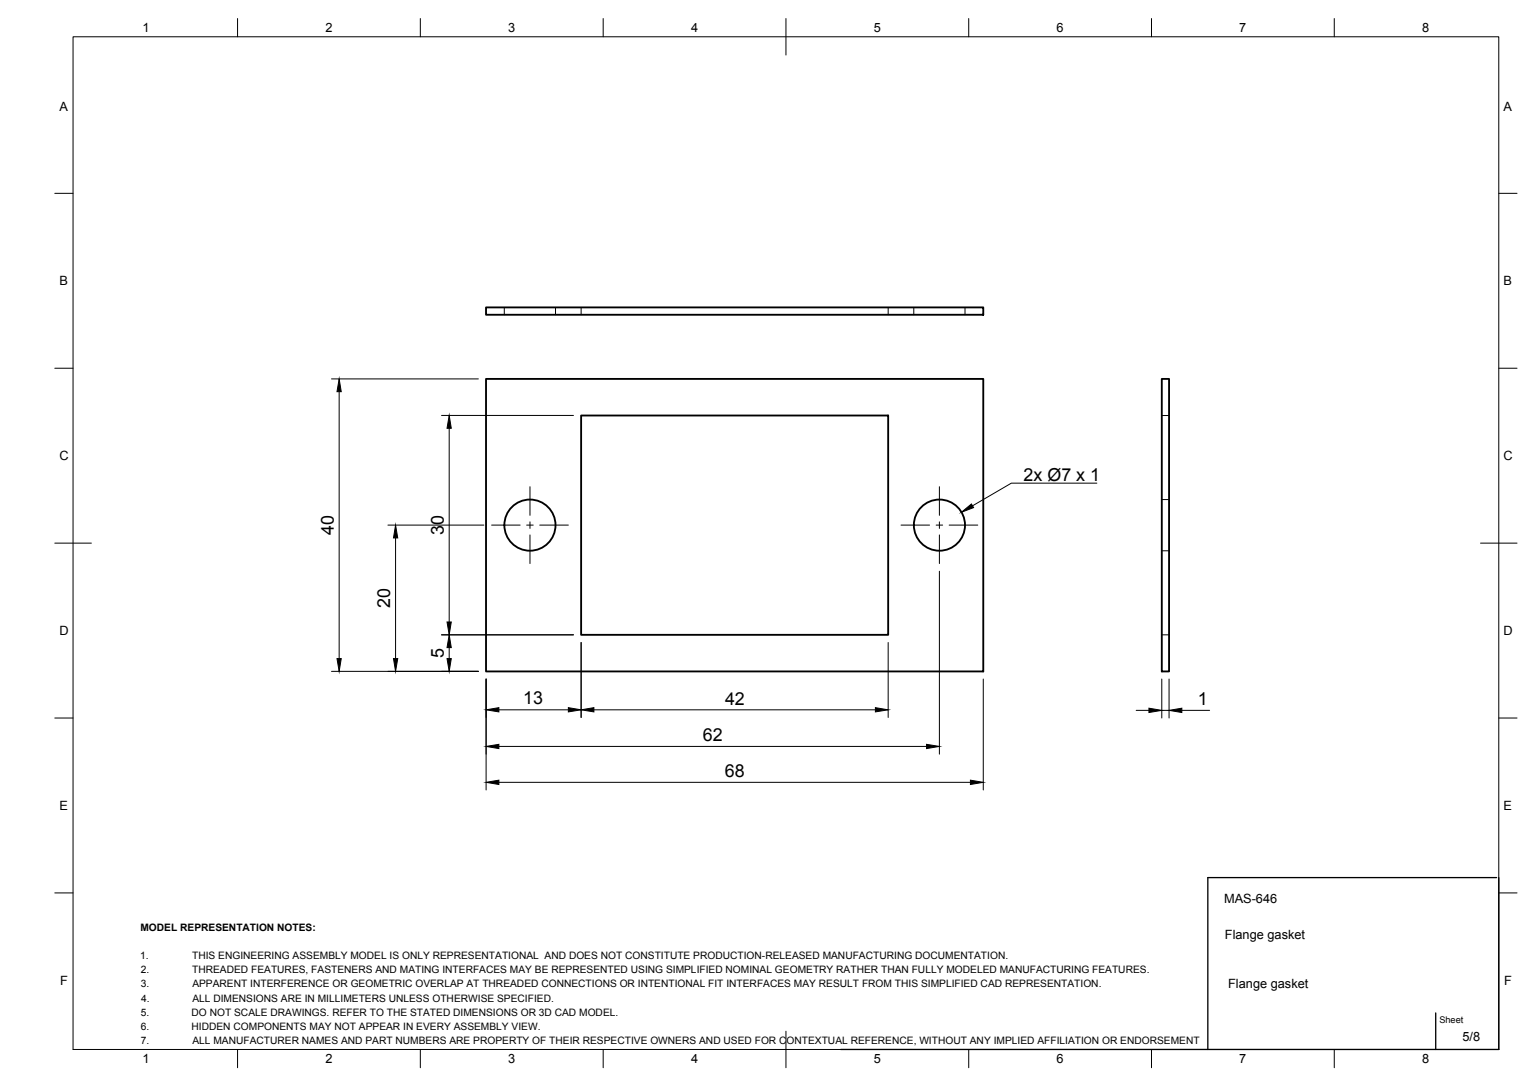
ISO-10303-21;
HEADER;
/* Generated by software containing ST-Developer
 * from STEP Tools, Inc. (www.steptools.com) 
 */

FILE_DESCRIPTION(
/* description */ ('Independent keyed three-contact power inlet for the IEC-connector des
ign category. Longer ground blade, retained contacts, wire termination
 holes and sealed bolted panel interface. Nominal custom interface; IE
C dimensional compatibility and electrical ratings are not assigned.'),

/* implementation_level */ '2;1');

FILE_NAME(
/* name */ 'Flange gasket.step',
/* time_stamp */ '2026-11-08T19:55:04-08:00',
/* author */ (''),
/* organization */ (''),
/* preprocessor_version */ 'ST-DEVELOPER v20.2',
/* originating_system */ 'Autodesk Translation Framework v15.17.0.0',
/* authorisation */ '');

FILE_SCHEMA (('AUTOMOTIVE_DESIGN { 1 0 10303 214 3 1 1 }'));
ENDSEC;

DATA;
#10=MECHANICAL_DESIGN_GEOMETRIC_PRESENTATION_REPRESENTATION('',(#111),#21880);
#91=SHAPE_REPRESENTATION_RELATIONSHIP('SRR','None',#21927,#101);
#101=ADVANCED_BREP_SHAPE_REPRESENTATION('',(#121),#21872);
#111=STYLED_ITEM('',(#21986),#121);
#121=MANIFOLD_SOLID_BREP('Body1',#6383);
#165=FACE_BOUND('',#890,.T.);
#166=FACE_BOUND('',#891,.T.);
#167=FACE_BOUND('',#892,.T.);
#168=FACE_BOUND('',#894,.T.);
#169=FACE_BOUND('',#895,.T.);
#170=FACE_BOUND('',#896,.T.);
#243=PLANE('',#6761);
#244=PLANE('',#6762);
#245=PLANE('',#6763);
#246=PLANE('',#6764);
#247=PLANE('',#6765);
#248=PLANE('',#6766);
#249=PLANE('',#6767);
#250=PLANE('',#6768);
#251=PLANE('',#6769);
#252=PLANE('',#6770);
#513=FACE_OUTER_BOUND('',#879,.T.);
#514=FACE_OUTER_BOUND('',#880,.T.);
#515=FACE_OUTER_BOUND('',#881,.T.);
#516=FACE_OUTER_BOUND('',#882,.T.);
#517=FACE_OUTER_BOUND('',#883,.T.);
#518=FACE_OUTER_BOUND('',#884,.T.);
#519=FACE_OUTER_BOUND('',#885,.T.);
#520=FACE_OUTER_BOUND('',#886,.T.);
#521=FACE_OUTER_BOUND('',#887,.T.);
#522=FACE_OUTER_BOUND('',#888,.T.);
#523=FACE_OUTER_BOUND('',#889,.T.);
#524=FACE_OUTER_BOUND('',#893,.T.);
#879=EDGE_LOOP('',(#5015,#5016,#5017,#5018));
#880=EDGE_LOOP('',(#5019,#5020,#5021,#5022));
#881=EDGE_LOOP('',(#5023,#5024,#5025,#5026));
#882=EDGE_LOOP('',(#5027,#5028,#5029,#5030));
#883=EDGE_LOOP('',(#5031,#5032,#5033,#5034));
#884=EDGE_LOOP('',(#5035,#5036,#5037,#5038));
#885=EDGE_LOOP('',(#5039,#5040,#5041,#5042));
#886=EDGE_LOOP('',(#5043,#5044,#5045,#5046));
#887=EDGE_LOOP('',(#5047,#5048,#5049,#5050));
#888=EDGE_LOOP('',(#5051,#5052,#5053,#5054));
#889=EDGE_LOOP('',(#5055,#5056,#5057,#5058));
#890=EDGE_LOOP('',(#5059));
#891=EDGE_LOOP('',(#5060));
#892=EDGE_LOOP('',(#5061,#5062,#5063,#5064));
#893=EDGE_LOOP('',(#5065,#5066,#5067,#5068));
#894=EDGE_LOOP('',(#5069));
#895=EDGE_LOOP('',(#5070));
#896=EDGE_LOOP('',(#5071,#5072,#5073,#5074));
#1124=CIRCLE('',#6756,3.5);
#1125=CIRCLE('',#6757,3.5);
#1126=CIRCLE('',#6759,3.5);
#1127=CIRCLE('',#6760,3.5);
#1761=LINE('',#16100,#2217);
#1762=LINE('',#16106,#2218);
#1763=LINE('',#16111,#2219);
#1764=LINE('',#16113,#2220);
#1765=LINE('',#16115,#2221);
#1766=LINE('',#16116,#2222);
#1767=LINE('',#16119,#2223);
#1768=LINE('',#16121,#2224);
#1769=LINE('',#16122,#2225);
#1770=LINE('',#16125,#2226);
#1771=LINE('',#16127,#2227);
#1772=LINE('',#16128,#2228);
#1773=LINE('',#16130,#2229);
#1774=LINE('',#16131,#2230);
#1775=LINE('',#16135,#2231);
#1776=LINE('',#16137,#2232);
#1777=LINE('',#16139,#2233);
#1778=LINE('',#16140,#2234);
#1779=LINE('',#16143,#2235);
#1780=LINE('',#16145,#2236);
#1781=LINE('',#16146,#2237);
#1782=LINE('',#16149,#2238);
#1783=LINE('',#16151,#2239);
#1784=LINE('',#16152,#2240);
#1785=LINE('',#16154,#2241);
#1786=LINE('',#16155,#2242);
#2217=VECTOR('',#7709,3.5);
#2218=VECTOR('',#7716,3.5);
#2219=VECTOR('',#7721,10.);
#2220=VECTOR('',#7722,10.);
#2221=VECTOR('',#7723,10.);
#2222=VECTOR('',#7724,10.);
#2223=VECTOR('',#7727,10.);
#2224=VECTOR('',#7728,10.);
#2225=VECTOR('',#7729,10.);
#2226=VECTOR('',#7732,10.);
#2227=VECTOR('',#7733,10.);
#2228=VECTOR('',#7734,10.);
#2229=VECTOR('',#7737,10.);
#2230=VECTOR('',#7738,10.);
#2231=VECTOR('',#7741,10.);
#2232=VECTOR('',#7742,10.);
#2233=VECTOR('',#7743,10.);
#2234=VECTOR('',#7744,10.);
#2235=VECTOR('',#7747,10.);
#2236=VECTOR('',#7748,10.);
#2237=VECTOR('',#7749,10.);
#2238=VECTOR('',#7752,10.);
#2239=VECTOR('',#7753,10.);
#2240=VECTOR('',#7754,10.);
#2241=VECTOR('',#7757,10.);
#2242=VECTOR('',#7758,10.);
#2775=VERTEX_POINT('',#16097);
#2776=VERTEX_POINT('',#16099);
#2777=VERTEX_POINT('',#16103);
#2778=VERTEX_POINT('',#16105);
#2779=VERTEX_POINT('',#16109);
#2780=VERTEX_POINT('',#16110);
#2781=VERTEX_POINT('',#16112);
#2782=VERTEX_POINT('',#16114);
#2783=VERTEX_POINT('',#16118);
#2784=VERTEX_POINT('',#16120);
#2785=VERTEX_POINT('',#16124);
#2786=VERTEX_POINT('',#16126);
#2787=VERTEX_POINT('',#16133);
#2788=VERTEX_POINT('',#16134);
#2789=VERTEX_POINT('',#16136);
#2790=VERTEX_POINT('',#16138);
#2791=VERTEX_POINT('',#16142);
#2792=VERTEX_POINT('',#16144);
#2793=VERTEX_POINT('',#16148);
#2794=VERTEX_POINT('',#16150);
#3567=EDGE_CURVE('',#2775,#2775,#1124,.T.);
#3568=EDGE_CURVE('',#2775,#2776,#1761,.T.);
#3569=EDGE_CURVE('',#2776,#2776,#1125,.T.);
#3570=EDGE_CURVE('',#2777,#2777,#1126,.T.);
#3571=EDGE_CURVE('',#2777,#2778,#1762,.T.);
#3572=EDGE_CURVE('',#2778,#2778,#1127,.T.);
#3573=EDGE_CURVE('',#2779,#2780,#1763,.T.);
#3574=EDGE_CURVE('',#2780,#2781,#1764,.T.);
#3575=EDGE_CURVE('',#2782,#2781,#1765,.T.);
#3576=EDGE_CURVE('',#2779,#2782,#1766,.T.);
#3577=EDGE_CURVE('',#2783,#2779,#1767,.T.);
#3578=EDGE_CURVE('',#2784,#2782,#1768,.T.);
#3579=EDGE_CURVE('',#2783,#2784,#1769,.T.);
#3580=EDGE_CURVE('',#2785,#2783,#1770,.T.);
#3581=EDGE_CURVE('',#2786,#2784,#1771,.T.);
#3582=EDGE_CURVE('',#2785,#2786,#1772,.T.);
#3583=EDGE_CURVE('',#2780,#2785,#1773,.T.);
#3584=EDGE_CURVE('',#2781,#2786,#1774,.T.);
#3585=EDGE_CURVE('',#2787,#2788,#1775,.T.);
#3586=EDGE_CURVE('',#2788,#2789,#1776,.T.);
#3587=EDGE_CURVE('',#2790,#2789,#1777,.T.);
#3588=EDGE_CURVE('',#2787,#2790,#1778,.T.);
#3589=EDGE_CURVE('',#2791,#2787,#1779,.T.);
#3590=EDGE_CURVE('',#2792,#2790,#1780,.T.);
#3591=EDGE_CURVE('',#2791,#2792,#1781,.T.);
#3592=EDGE_CURVE('',#2793,#2791,#1782,.T.);
#3593=EDGE_CURVE('',#2794,#2792,#1783,.T.);
#3594=EDGE_CURVE('',#2793,#2794,#1784,.T.);
#3595=EDGE_CURVE('',#2788,#2793,#1785,.T.);
#3596=EDGE_CURVE('',#2789,#2794,#1786,.T.);
#5015=ORIENTED_EDGE('',*,*,#3567,.F.);
#5016=ORIENTED_EDGE('',*,*,#3568,.T.);
#5017=ORIENTED_EDGE('',*,*,#3569,.F.);
#5018=ORIENTED_EDGE('',*,*,#3568,.F.);
#5019=ORIENTED_EDGE('',*,*,#3570,.F.);
#5020=ORIENTED_EDGE('',*,*,#3571,.T.);
#5021=ORIENTED_EDGE('',*,*,#3572,.F.);
#5022=ORIENTED_EDGE('',*,*,#3571,.F.);
#5023=ORIENTED_EDGE('',*,*,#3573,.T.);
#5024=ORIENTED_EDGE('',*,*,#3574,.T.);
#5025=ORIENTED_EDGE('',*,*,#3575,.F.);
#5026=ORIENTED_EDGE('',*,*,#3576,.F.);
#5027=ORIENTED_EDGE('',*,*,#3577,.T.);
#5028=ORIENTED_EDGE('',*,*,#3576,.T.);
#5029=ORIENTED_EDGE('',*,*,#3578,.F.);
#5030=ORIENTED_EDGE('',*,*,#3579,.F.);
#5031=ORIENTED_EDGE('',*,*,#3580,.T.);
#5032=ORIENTED_EDGE('',*,*,#3579,.T.);
#5033=ORIENTED_EDGE('',*,*,#3581,.F.);
#5034=ORIENTED_EDGE('',*,*,#3582,.F.);
#5035=ORIENTED_EDGE('',*,*,#3583,.T.);
#5036=ORIENTED_EDGE('',*,*,#3582,.T.);
#5037=ORIENTED_EDGE('',*,*,#3584,.F.);
#5038=ORIENTED_EDGE('',*,*,#3574,.F.);
#5039=ORIENTED_EDGE('',*,*,#3585,.T.);
#5040=ORIENTED_EDGE('',*,*,#3586,.T.);
#5041=ORIENTED_EDGE('',*,*,#3587,.F.);
#5042=ORIENTED_EDGE('',*,*,#3588,.F.);
#5043=ORIENTED_EDGE('',*,*,#3589,.T.);
#5044=ORIENTED_EDGE('',*,*,#3588,.T.);
#5045=ORIENTED_EDGE('',*,*,#3590,.F.);
#5046=ORIENTED_EDGE('',*,*,#3591,.F.);
#5047=ORIENTED_EDGE('',*,*,#3592,.T.);
#5048=ORIENTED_EDGE('',*,*,#3591,.T.);
#5049=ORIENTED_EDGE('',*,*,#3593,.F.);
#5050=ORIENTED_EDGE('',*,*,#3594,.F.);
#5051=ORIENTED_EDGE('',*,*,#3595,.T.);
#5052=ORIENTED_EDGE('',*,*,#3594,.T.);
#5053=ORIENTED_EDGE('',*,*,#3596,.F.);
#5054=ORIENTED_EDGE('',*,*,#3586,.F.);
#5055=ORIENTED_EDGE('',*,*,#3596,.T.);
#5056=ORIENTED_EDGE('',*,*,#3593,.T.);
#5057=ORIENTED_EDGE('',*,*,#3590,.T.);
#5058=ORIENTED_EDGE('',*,*,#3587,.T.);
#5059=ORIENTED_EDGE('',*,*,#3567,.T.);
#5060=ORIENTED_EDGE('',*,*,#3570,.T.);
#5061=ORIENTED_EDGE('',*,*,#3584,.T.);
#5062=ORIENTED_EDGE('',*,*,#3581,.T.);
#5063=ORIENTED_EDGE('',*,*,#3578,.T.);
#5064=ORIENTED_EDGE('',*,*,#3575,.T.);
#5065=ORIENTED_EDGE('',*,*,#3595,.F.);
#5066=ORIENTED_EDGE('',*,*,#3585,.F.);
#5067=ORIENTED_EDGE('',*,*,#3589,.F.);
#5068=ORIENTED_EDGE('',*,*,#3592,.F.);
#5069=ORIENTED_EDGE('',*,*,#3569,.T.);
#5070=ORIENTED_EDGE('',*,*,#3572,.T.);
#5071=ORIENTED_EDGE('',*,*,#3583,.F.);
#5072=ORIENTED_EDGE('',*,*,#3573,.F.);
#5073=ORIENTED_EDGE('',*,*,#3577,.F.);
#5074=ORIENTED_EDGE('',*,*,#3580,.F.);
#5957=CYLINDRICAL_SURFACE('',#6755,3.5);
#5958=CYLINDRICAL_SURFACE('',#6758,3.5);
#6225=ADVANCED_FACE('',(#513),#5957,.F.);
#6226=ADVANCED_FACE('',(#514),#5958,.F.);
#6227=ADVANCED_FACE('',(#515),#243,.T.);
#6228=ADVANCED_FACE('',(#516),#244,.T.);
#6229=ADVANCED_FACE('',(#517),#245,.T.);
#6230=ADVANCED_FACE('',(#518),#246,.T.);
#6231=ADVANCED_FACE('',(#519),#247,.T.);
#6232=ADVANCED_FACE('',(#520),#248,.T.);
#6233=ADVANCED_FACE('',(#521),#249,.T.);
#6234=ADVANCED_FACE('',(#522),#250,.T.);
#6235=ADVANCED_FACE('',(#523,#165,#166,#167),#251,.T.);
#6236=ADVANCED_FACE('',(#524,#168,#169,#170),#252,.F.);
#6383=CLOSED_SHELL('',(#6225,#6226,#6227,#6228,#6229,#6230,#6231,#6232,
#6233,#6234,#6235,#6236));
#6754=AXIS2_PLACEMENT_3D('',#16095,#7703,#7704);
#6755=AXIS2_PLACEMENT_3D('',#16096,#7705,#7706);
#6756=AXIS2_PLACEMENT_3D('',#16098,#7707,#7708);
#6757=AXIS2_PLACEMENT_3D('',#16101,#7710,#7711);
#6758=AXIS2_PLACEMENT_3D('',#16102,#7712,#7713);
#6759=AXIS2_PLACEMENT_3D('',#16104,#7714,#7715);
#6760=AXIS2_PLACEMENT_3D('',#16107,#7717,#7718);
#6761=AXIS2_PLACEMENT_3D('',#16108,#7719,#7720);
#6762=AXIS2_PLACEMENT_3D('',#16117,#7725,#7726);
#6763=AXIS2_PLACEMENT_3D('',#16123,#7730,#7731);
#6764=AXIS2_PLACEMENT_3D('',#16129,#7735,#7736);
#6765=AXIS2_PLACEMENT_3D('',#16132,#7739,#7740);
#6766=AXIS2_PLACEMENT_3D('',#16141,#7745,#7746);
#6767=AXIS2_PLACEMENT_3D('',#16147,#7750,#7751);
#6768=AXIS2_PLACEMENT_3D('',#16153,#7755,#7756);
#6769=AXIS2_PLACEMENT_3D('',#16156,#7759,#7760);
#6770=AXIS2_PLACEMENT_3D('',#16157,#7761,#7762);
#7703=DIRECTION('axis',(0.,0.,1.));
#7704=DIRECTION('refdir',(1.,0.,0.));
#7705=DIRECTION('center_axis',(0.,0.,-1.));
#7706=DIRECTION('ref_axis',(1.,0.,0.));
#7707=DIRECTION('center_axis',(0.,0.,-1.));
#7708=DIRECTION('ref_axis',(1.,0.,0.));
#7709=DIRECTION('',(0.,0.,-1.));
#7710=DIRECTION('center_axis',(0.,0.,1.));
#7711=DIRECTION('ref_axis',(1.,0.,0.));
#7712=DIRECTION('center_axis',(0.,0.,-1.));
#7713=DIRECTION('ref_axis',(1.,0.,0.));
#7714=DIRECTION('center_axis',(0.,0.,-1.));
#7715=DIRECTION('ref_axis',(1.,0.,0.));
#7716=DIRECTION('',(0.,0.,-1.));
#7717=DIRECTION('center_axis',(0.,0.,1.));
#7718=DIRECTION('ref_axis',(1.,0.,0.));
#7719=DIRECTION('center_axis',(0.,1.,0.));
#7720=DIRECTION('ref_axis',(-1.,0.,0.));
#7721=DIRECTION('',(-1.,0.,0.));
#7722=DIRECTION('',(0.,0.,1.));
#7723=DIRECTION('',(-1.,0.,0.));
#7724=DIRECTION('',(0.,0.,1.));
#7725=DIRECTION('center_axis',(-1.,0.,0.));
#7726=DIRECTION('ref_axis',(0.,-1.,0.));
#7727=DIRECTION('',(0.,-1.,0.));
#7728=DIRECTION('',(0.,-1.,0.));
#7729=DIRECTION('',(0.,0.,1.));
#7730=DIRECTION('center_axis',(0.,-1.,0.));
#7731=DIRECTION('ref_axis',(1.,0.,0.));
#7732=DIRECTION('',(1.,0.,0.));
#7733=DIRECTION('',(1.,0.,0.));
#7734=DIRECTION('',(0.,0.,1.));
#7735=DIRECTION('center_axis',(1.,0.,0.));
#7736=DIRECTION('ref_axis',(0.,1.,0.));
#7737=DIRECTION('',(0.,1.,0.));
#7738=DIRECTION('',(0.,1.,0.));
#7739=DIRECTION('center_axis',(0.,1.,0.));
#7740=DIRECTION('ref_axis',(-1.,0.,0.));
#7741=DIRECTION('',(-1.,0.,0.));
#7742=DIRECTION('',(0.,0.,1.));
#7743=DIRECTION('',(-1.,0.,0.));
#7744=DIRECTION('',(0.,0.,1.));
#7745=DIRECTION('center_axis',(1.,0.,0.));
#7746=DIRECTION('ref_axis',(0.,1.,0.));
#7747=DIRECTION('',(0.,1.,0.));
#7748=DIRECTION('',(0.,1.,0.));
#7749=DIRECTION('',(0.,0.,1.));
#7750=DIRECTION('center_axis',(0.,-1.,0.));
#7751=DIRECTION('ref_axis',(1.,0.,0.));
#7752=DIRECTION('',(1.,0.,0.));
#7753=DIRECTION('',(1.,0.,0.));
#7754=DIRECTION('',(0.,0.,1.));
#7755=DIRECTION('center_axis',(-1.,0.,0.));
#7756=DIRECTION('ref_axis',(0.,-1.,0.));
#7757=DIRECTION('',(0.,-1.,0.));
#7758=DIRECTION('',(0.,-1.,0.));
#7759=DIRECTION('center_axis',(0.,0.,1.));
#7760=DIRECTION('ref_axis',(1.,0.,0.));
#7761=DIRECTION('center_axis',(0.,0.,1.));
#7762=DIRECTION('ref_axis',(1.,0.,0.));
#16095=CARTESIAN_POINT('',(0.,0.,0.));
#16096=CARTESIAN_POINT('Origin',(-28.,0.,0.5));
#16097=CARTESIAN_POINT('',(-31.5,4.28626379701574E-16,1.));
#16098=CARTESIAN_POINT('Origin',(-28.,0.,1.));
#16099=CARTESIAN_POINT('',(-31.5,4.28626379701574E-16,0.));
#16100=CARTESIAN_POINT('',(-31.5,4.28626379701574E-16,0.5));
#16101=CARTESIAN_POINT('Origin',(-28.,0.,0.));
#16102=CARTESIAN_POINT('Origin',(28.,0.,0.5));
#16103=CARTESIAN_POINT('',(24.5,4.28626379701574E-16,1.));
#16104=CARTESIAN_POINT('Origin',(28.,0.,1.));
#16105=CARTESIAN_POINT('',(24.5,4.28626379701574E-16,0.));
#16106=CARTESIAN_POINT('',(24.5,4.28626379701574E-16,0.5));
#16107=CARTESIAN_POINT('Origin',(28.,0.,0.));
#16108=CARTESIAN_POINT('Origin',(21.,-15.,0.));
#16109=CARTESIAN_POINT('',(21.,-15.,0.));
#16110=CARTESIAN_POINT('',(-21.,-15.,0.));
#16111=CARTESIAN_POINT('',(-21.,-15.,0.));
#16112=CARTESIAN_POINT('',(-21.,-15.,1.));
#16113=CARTESIAN_POINT('',(-21.,-15.,0.));
#16114=CARTESIAN_POINT('',(21.,-15.,1.));
#16115=CARTESIAN_POINT('',(-21.,-15.,1.));
#16116=CARTESIAN_POINT('',(21.,-15.,0.));
#16117=CARTESIAN_POINT('Origin',(21.,15.,0.));
#16118=CARTESIAN_POINT('',(21.,15.,0.));
#16119=CARTESIAN_POINT('',(21.,-15.,0.));
#16120=CARTESIAN_POINT('',(21.,15.,1.));
#16121=CARTESIAN_POINT('',(21.,-15.,1.));
#16122=CARTESIAN_POINT('',(21.,15.,0.));
#16123=CARTESIAN_POINT('Origin',(-21.,15.,0.));
#16124=CARTESIAN_POINT('',(-21.,15.,0.));
#16125=CARTESIAN_POINT('',(21.,15.,0.));
#16126=CARTESIAN_POINT('',(-21.,15.,1.));
#16127=CARTESIAN_POINT('',(21.,15.,1.));
#16128=CARTESIAN_POINT('',(-21.,15.,0.));
#16129=CARTESIAN_POINT('Origin',(-21.,-15.,0.));
#16130=CARTESIAN_POINT('',(-21.,15.,0.));
#16131=CARTESIAN_POINT('',(-21.,15.,1.));
#16132=CARTESIAN_POINT('Origin',(34.,20.,0.));
#16133=CARTESIAN_POINT('',(34.,20.,0.));
#16134=CARTESIAN_POINT('',(-34.,20.,0.));
#16135=CARTESIAN_POINT('',(34.,20.,0.));
#16136=CARTESIAN_POINT('',(-34.,20.,1.));
#16137=CARTESIAN_POINT('',(-34.,20.,0.));
#16138=CARTESIAN_POINT('',(34.,20.,1.));
#16139=CARTESIAN_POINT('',(34.,20.,1.));
#16140=CARTESIAN_POINT('',(34.,20.,0.));
#16141=CARTESIAN_POINT('Origin',(34.,-20.,0.));
#16142=CARTESIAN_POINT('',(34.,-20.,0.));
#16143=CARTESIAN_POINT('',(34.,-20.,0.));
#16144=CARTESIAN_POINT('',(34.,-20.,1.));
#16145=CARTESIAN_POINT('',(34.,-20.,1.));
#16146=CARTESIAN_POINT('',(34.,-20.,0.));
#16147=CARTESIAN_POINT('Origin',(-34.,-20.,0.));
#16148=CARTESIAN_POINT('',(-34.,-20.,0.));
#16149=CARTESIAN_POINT('',(-34.,-20.,0.));
#16150=CARTESIAN_POINT('',(-34.,-20.,1.));
#16151=CARTESIAN_POINT('',(-34.,-20.,1.));
#16152=CARTESIAN_POINT('',(-34.,-20.,0.));
#16153=CARTESIAN_POINT('Origin',(-34.,20.,0.));
#16154=CARTESIAN_POINT('',(-34.,20.,0.));
#16155=CARTESIAN_POINT('',(-34.,20.,1.));
#16156=CARTESIAN_POINT('Origin',(0.,0.,1.));
#16157=CARTESIAN_POINT('Origin',(0.,0.,0.));
#21860=UNCERTAINTY_MEASURE_WITH_UNIT(LENGTH_MEASURE(0.01),#21881,
'DISTANCE_ACCURACY_VALUE',
'Maximum model space distance between geometric entities at asserted c
onnectivities');
#21868=UNCERTAINTY_MEASURE_WITH_UNIT(LENGTH_MEASURE(0.01),#21881,
'DISTANCE_ACCURACY_VALUE',
'Maximum model space distance between geometric entities at asserted c
onnectivities');
#21872=(
GEOMETRIC_REPRESENTATION_CONTEXT(3)
GLOBAL_UNCERTAINTY_ASSIGNED_CONTEXT((#21860))
GLOBAL_UNIT_ASSIGNED_CONTEXT((#21881,#21883,#21884))
REPRESENTATION_CONTEXT('','3D')
);
#21880=(
GEOMETRIC_REPRESENTATION_CONTEXT(3)
GLOBAL_UNCERTAINTY_ASSIGNED_CONTEXT((#21868))
GLOBAL_UNIT_ASSIGNED_CONTEXT((#21881,#21883,#21884))
REPRESENTATION_CONTEXT('','3D')
);
#21881=(
LENGTH_UNIT()
NAMED_UNIT(*)
SI_UNIT(.MILLI.,.METRE.)
);
#21883=(
NAMED_UNIT(*)
PLANE_ANGLE_UNIT()
SI_UNIT($,.RADIAN.)
);
#21884=(
NAMED_UNIT(*)
SI_UNIT($,.STERADIAN.)
SOLID_ANGLE_UNIT()
);
#21888=SHAPE_DEFINITION_REPRESENTATION(#21899,#21927);
#21899=PRODUCT_DEFINITION_SHAPE('',$,#21939);
#21927=SHAPE_REPRESENTATION('',(#6754),#21872);
#21935=PRODUCT_DEFINITION_CONTEXT('part definition',#21970,'design');
#21939=PRODUCT_DEFINITION('Flange gasket','Flange gasket',#21950,#21935);
#21950=PRODUCT_DEFINITION_FORMATION('',$,#21975);
#21970=APPLICATION_CONTEXT(
'Core Data for Automotive Mechanical Design Process');
#21971=PRODUCT_CONTEXT('part definition',#21970,'mechanical');
#21975=PRODUCT('Flange gasket','Flange gasket',$,(#21971));
#21986=PRESENTATION_STYLE_ASSIGNMENT((#21992));
#21992=SURFACE_STYLE_USAGE(.BOTH.,#21998);
#21998=SURFACE_SIDE_STYLE('',(#22004));
#22004=SURFACE_STYLE_FILL_AREA(#22010);
#22010=FILL_AREA_STYLE('Dark gray',(#22016));
#22016=FILL_AREA_STYLE_COLOUR('Dark gray',#22022);
#22022=COLOUR_RGB('Dark gray',0.250980392156863,0.282352941176471,0.32156862745098);
ENDSEC;
END-ISO-10303-21;
